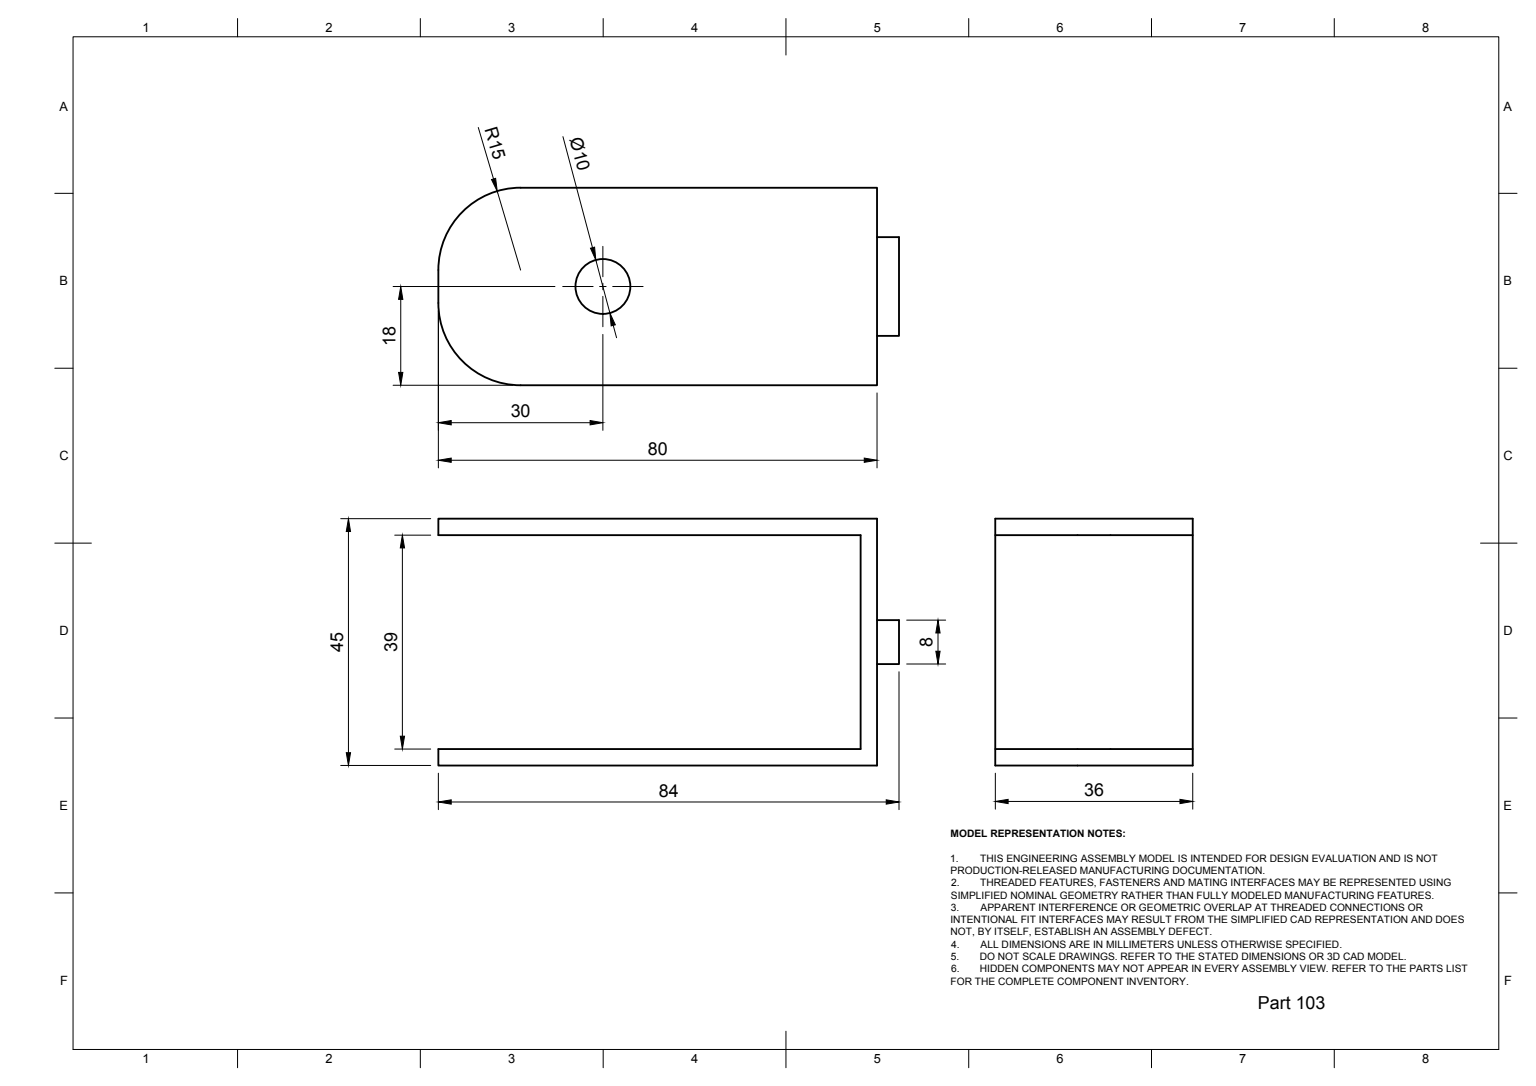
ISO-10303-21;
HEADER;
/* Generated by software containing ST-Developer
 * from STEP Tools, Inc. (www.steptools.com) 
 */

FILE_DESCRIPTION(
/* description */ (''),
/* implementation_level */ '2;1');

FILE_NAME(
/* name */ 'Part 103.step',
/* time_stamp */ '2026-10-07T11:02:43-07:00',
/* author */ (''),
/* organization */ (''),
/* preprocessor_version */ 'ST-DEVELOPER v20.2',
/* originating_system */ 'Autodesk Translation Framework v15.15.0.0',
/* authorisation */ '');

FILE_SCHEMA (('AUTOMOTIVE_DESIGN { 1 0 10303 214 3 1 1 }'));
ENDSEC;

DATA;
#10=MECHANICAL_DESIGN_GEOMETRIC_PRESENTATION_REPRESENTATION('',(#72),#5505);
#58=SHAPE_REPRESENTATION_RELATIONSHIP('SRR','None',#5543,#65);
#65=ADVANCED_BREP_SHAPE_REPRESENTATION('',(#79),#5504);
#72=STYLED_ITEM('',(#5587),#79);
#79=MANIFOLD_SOLID_BREP('Body1',#3299);
#108=FACE_BOUND('',#577,.T.);
#109=FACE_BOUND('',#579,.T.);
#110=FACE_BOUND('',#582,.T.);
#111=FACE_BOUND('',#584,.T.);
#112=FACE_BOUND('',#586,.T.);
#147=CYLINDRICAL_SURFACE('',#3629,15.);
#148=CYLINDRICAL_SURFACE('',#3630,15.);
#149=CYLINDRICAL_SURFACE('',#3631,15.);
#150=CYLINDRICAL_SURFACE('',#3632,15.);
#151=CYLINDRICAL_SURFACE('',#3633,5.);
#152=CYLINDRICAL_SURFACE('',#3634,5.);
#224=CIRCLE('',#3604,15.);
#225=CIRCLE('',#3605,15.);
#226=CIRCLE('',#3606,5.);
#227=CIRCLE('',#3608,15.);
#228=CIRCLE('',#3609,15.);
#229=CIRCLE('',#3610,5.);
#230=CIRCLE('',#3613,15.);
#231=CIRCLE('',#3614,15.);
#232=CIRCLE('',#3615,5.);
#233=CIRCLE('',#3617,15.);
#234=CIRCLE('',#3618,15.);
#235=CIRCLE('',#3619,5.);
#381=FACE_OUTER_BOUND('',#575,.T.);
#382=FACE_OUTER_BOUND('',#576,.T.);
#383=FACE_OUTER_BOUND('',#578,.T.);
#384=FACE_OUTER_BOUND('',#580,.T.);
#385=FACE_OUTER_BOUND('',#581,.T.);
#386=FACE_OUTER_BOUND('',#583,.T.);
#387=FACE_OUTER_BOUND('',#585,.T.);
#388=FACE_OUTER_BOUND('',#587,.T.);
#389=FACE_OUTER_BOUND('',#588,.T.);
#390=FACE_OUTER_BOUND('',#589,.T.);
#391=FACE_OUTER_BOUND('',#590,.T.);
#392=FACE_OUTER_BOUND('',#591,.T.);
#393=FACE_OUTER_BOUND('',#592,.T.);
#394=FACE_OUTER_BOUND('',#593,.T.);
#395=FACE_OUTER_BOUND('',#594,.T.);
#396=FACE_OUTER_BOUND('',#595,.T.);
#397=FACE_OUTER_BOUND('',#596,.T.);
#398=FACE_OUTER_BOUND('',#597,.T.);
#399=FACE_OUTER_BOUND('',#598,.T.);
#400=FACE_OUTER_BOUND('',#599,.T.);
#401=FACE_OUTER_BOUND('',#600,.T.);
#575=EDGE_LOOP('',(#2894,#2895,#2896,#2897));
#576=EDGE_LOOP('',(#2898,#2899,#2900,#2901,#2902,#2903));
#577=EDGE_LOOP('',(#2904));
#578=EDGE_LOOP('',(#2905,#2906,#2907,#2908,#2909,#2910));
#579=EDGE_LOOP('',(#2911));
#580=EDGE_LOOP('',(#2912,#2913,#2914,#2915));
#581=EDGE_LOOP('',(#2916,#2917,#2918,#2919,#2920,#2921));
#582=EDGE_LOOP('',(#2922));
#583=EDGE_LOOP('',(#2923,#2924,#2925,#2926,#2927,#2928));
#584=EDGE_LOOP('',(#2929));
#585=EDGE_LOOP('',(#2930,#2931,#2932,#2933));
#586=EDGE_LOOP('',(#2934,#2935,#2936,#2937));
#587=EDGE_LOOP('',(#2938,#2939,#2940,#2941,#2942,#2943,#2944,#2945));
#588=EDGE_LOOP('',(#2946,#2947,#2948,#2949,#2950,#2951,#2952,#2953));
#589=EDGE_LOOP('',(#2954,#2955,#2956,#2957));
#590=EDGE_LOOP('',(#2958,#2959,#2960,#2961));
#591=EDGE_LOOP('',(#2962,#2963,#2964,#2965));
#592=EDGE_LOOP('',(#2966,#2967,#2968,#2969));
#593=EDGE_LOOP('',(#2970,#2971,#2972,#2973));
#594=EDGE_LOOP('',(#2974,#2975,#2976,#2977));
#595=EDGE_LOOP('',(#2978,#2979,#2980,#2981));
#596=EDGE_LOOP('',(#2982,#2983,#2984,#2985));
#597=EDGE_LOOP('',(#2986,#2987,#2988,#2989));
#598=EDGE_LOOP('',(#2990,#2991,#2992,#2993));
#599=EDGE_LOOP('',(#2994,#2995,#2996,#2997));
#600=EDGE_LOOP('',(#2998,#2999,#3000,#3001));
#929=LINE('',#5370,#1299);
#930=LINE('',#5372,#1300);
#931=LINE('',#5374,#1301);
#932=LINE('',#5375,#1302);
#933=LINE('',#5379,#1303);
#934=LINE('',#5384,#1304);
#935=LINE('',#5385,#1305);
#936=LINE('',#5393,#1306);
#937=LINE('',#5395,#1307);
#938=LINE('',#5397,#1308);
#939=LINE('',#5400,#1309);
#940=LINE('',#5405,#1310);
#941=LINE('',#5407,#1311);
#942=LINE('',#5408,#1312);
#943=LINE('',#5413,#1313);
#944=LINE('',#5415,#1314);
#945=LINE('',#5417,#1315);
#946=LINE('',#5427,#1316);
#947=LINE('',#5429,#1317);
#948=LINE('',#5430,#1318);
#949=LINE('',#5434,#1319);
#950=LINE('',#5435,#1320);
#951=LINE('',#5438,#1321);
#952=LINE('',#5440,#1322);
#953=LINE('',#5442,#1323);
#954=LINE('',#5443,#1324);
#955=LINE('',#5445,#1325);
#956=LINE('',#5446,#1326);
#957=LINE('',#5447,#1327);
#958=LINE('',#5449,#1328);
#959=LINE('',#5450,#1329);
#960=LINE('',#5451,#1330);
#961=LINE('',#5455,#1331);
#962=LINE('',#5457,#1332);
#963=LINE('',#5458,#1333);
#964=LINE('',#5461,#1334);
#965=LINE('',#5462,#1335);
#966=LINE('',#5465,#1336);
#967=LINE('',#5466,#1337);
#968=LINE('',#5468,#1338);
#969=LINE('',#5475,#1339);
#970=LINE('',#5477,#1340);
#1299=VECTOR('',#4423,1000.);
#1300=VECTOR('',#4424,1000.);
#1301=VECTOR('',#4425,1000.);
#1302=VECTOR('',#4426,1000.);
#1303=VECTOR('',#4429,1000.);
#1304=VECTOR('',#4434,1000.);
#1305=VECTOR('',#4435,1000.);
#1306=VECTOR('',#4442,1000.);
#1307=VECTOR('',#4443,1000.);
#1308=VECTOR('',#4444,1000.);
#1309=VECTOR('',#4447,1000.);
#1310=VECTOR('',#4452,1000.);
#1311=VECTOR('',#4453,1000.);
#1312=VECTOR('',#4454,1000.);
#1313=VECTOR('',#4459,1000.);
#1314=VECTOR('',#4460,1000.);
#1315=VECTOR('',#4461,1000.);
#1316=VECTOR('',#4472,1000.);
#1317=VECTOR('',#4473,1000.);
#1318=VECTOR('',#4474,1000.);
#1319=VECTOR('',#4479,1000.);
#1320=VECTOR('',#4480,1000.);
#1321=VECTOR('',#4481,1000.);
#1322=VECTOR('',#4482,1000.);
#1323=VECTOR('',#4483,1000.);
#1324=VECTOR('',#4484,1000.);
#1325=VECTOR('',#4487,1000.);
#1326=VECTOR('',#4488,1000.);
#1327=VECTOR('',#4489,1000.);
#1328=VECTOR('',#4492,1000.);
#1329=VECTOR('',#4493,1000.);
#1330=VECTOR('',#4494,1000.);
#1331=VECTOR('',#4499,1000.);
#1332=VECTOR('',#4500,1000.);
#1333=VECTOR('',#4501,1000.);
#1334=VECTOR('',#4504,1000.);
#1335=VECTOR('',#4505,1000.);
#1336=VECTOR('',#4508,1000.);
#1337=VECTOR('',#4509,1000.);
#1338=VECTOR('',#4512,1000.);
#1339=VECTOR('',#4525,5.);
#1340=VECTOR('',#4528,5.);
#1607=VERTEX_POINT('',#5368);
#1608=VERTEX_POINT('',#5369);
#1609=VERTEX_POINT('',#5371);
#1610=VERTEX_POINT('',#5373);
#1611=VERTEX_POINT('',#5377);
#1612=VERTEX_POINT('',#5378);
#1613=VERTEX_POINT('',#5381);
#1614=VERTEX_POINT('',#5383);
#1615=VERTEX_POINT('',#5386);
#1616=VERTEX_POINT('',#5389);
#1617=VERTEX_POINT('',#5390);
#1618=VERTEX_POINT('',#5392);
#1619=VERTEX_POINT('',#5394);
#1620=VERTEX_POINT('',#5396);
#1621=VERTEX_POINT('',#5398);
#1622=VERTEX_POINT('',#5401);
#1623=VERTEX_POINT('',#5404);
#1624=VERTEX_POINT('',#5406);
#1625=VERTEX_POINT('',#5410);
#1626=VERTEX_POINT('',#5412);
#1627=VERTEX_POINT('',#5414);
#1628=VERTEX_POINT('',#5416);
#1629=VERTEX_POINT('',#5419);
#1630=VERTEX_POINT('',#5422);
#1631=VERTEX_POINT('',#5424);
#1632=VERTEX_POINT('',#5426);
#1633=VERTEX_POINT('',#5428);
#1634=VERTEX_POINT('',#5431);
#1635=VERTEX_POINT('',#5436);
#1636=VERTEX_POINT('',#5437);
#1637=VERTEX_POINT('',#5439);
#1638=VERTEX_POINT('',#5441);
#1639=VERTEX_POINT('',#5454);
#1640=VERTEX_POINT('',#5456);
#1641=VERTEX_POINT('',#5460);
#1642=VERTEX_POINT('',#5464);
#2042=EDGE_CURVE('',#1607,#1608,#929,.T.);
#2043=EDGE_CURVE('',#1608,#1609,#930,.T.);
#2044=EDGE_CURVE('',#1610,#1609,#931,.T.);
#2045=EDGE_CURVE('',#1607,#1610,#932,.T.);
#2046=EDGE_CURVE('',#1611,#1612,#933,.T.);
#2047=EDGE_CURVE('',#1611,#1610,#224,.T.);
#2048=EDGE_CURVE('',#1609,#1613,#225,.T.);
#2049=EDGE_CURVE('',#1613,#1614,#934,.T.);
#2050=EDGE_CURVE('',#1612,#1614,#935,.T.);
#2051=EDGE_CURVE('',#1615,#1615,#226,.T.);
#2052=EDGE_CURVE('',#1616,#1617,#227,.T.);
#2053=EDGE_CURVE('',#1616,#1618,#936,.T.);
#2054=EDGE_CURVE('',#1618,#1619,#937,.T.);
#2055=EDGE_CURVE('',#1620,#1619,#938,.T.);
#2056=EDGE_CURVE('',#1621,#1620,#228,.T.);
#2057=EDGE_CURVE('',#1617,#1621,#939,.T.);
#2058=EDGE_CURVE('',#1622,#1622,#229,.T.);
#2059=EDGE_CURVE('',#1621,#1623,#940,.T.);
#2060=EDGE_CURVE('',#1624,#1623,#941,.T.);
#2061=EDGE_CURVE('',#1617,#1624,#942,.T.);
#2062=EDGE_CURVE('',#1607,#1625,#230,.T.);
#2063=EDGE_CURVE('',#1626,#1625,#943,.T.);
#2064=EDGE_CURVE('',#1627,#1626,#944,.T.);
#2065=EDGE_CURVE('',#1628,#1627,#945,.T.);
#2066=EDGE_CURVE('',#1628,#1608,#231,.T.);
#2067=EDGE_CURVE('',#1629,#1629,#232,.T.);
#2068=EDGE_CURVE('',#1624,#1630,#233,.T.);
#2069=EDGE_CURVE('',#1631,#1623,#234,.T.);
#2070=EDGE_CURVE('',#1631,#1632,#946,.T.);
#2071=EDGE_CURVE('',#1632,#1633,#947,.T.);
#2072=EDGE_CURVE('',#1633,#1630,#948,.T.);
#2073=EDGE_CURVE('',#1634,#1634,#235,.T.);
#2074=EDGE_CURVE('',#1614,#1619,#949,.T.);
#2075=EDGE_CURVE('',#1612,#1618,#950,.T.);
#2076=EDGE_CURVE('',#1635,#1636,#951,.T.);
#2077=EDGE_CURVE('',#1635,#1637,#952,.T.);
#2078=EDGE_CURVE('',#1637,#1638,#953,.T.);
#2079=EDGE_CURVE('',#1636,#1638,#954,.T.);
#2080=EDGE_CURVE('',#1620,#1631,#955,.T.);
#2081=EDGE_CURVE('',#1628,#1613,#956,.T.);
#2082=EDGE_CURVE('',#1632,#1627,#957,.T.);
#2083=EDGE_CURVE('',#1616,#1630,#958,.T.);
#2084=EDGE_CURVE('',#1626,#1633,#959,.T.);
#2085=EDGE_CURVE('',#1625,#1611,#960,.T.);
#2086=EDGE_CURVE('',#1639,#1636,#961,.T.);
#2087=EDGE_CURVE('',#1640,#1639,#962,.T.);
#2088=EDGE_CURVE('',#1640,#1635,#963,.T.);
#2089=EDGE_CURVE('',#1641,#1638,#964,.T.);
#2090=EDGE_CURVE('',#1639,#1641,#965,.T.);
#2091=EDGE_CURVE('',#1642,#1637,#966,.T.);
#2092=EDGE_CURVE('',#1642,#1641,#967,.T.);
#2093=EDGE_CURVE('',#1640,#1642,#968,.T.);
#2094=EDGE_CURVE('',#1622,#1634,#969,.T.);
#2095=EDGE_CURVE('',#1629,#1615,#970,.T.);
#2894=ORIENTED_EDGE('',*,*,#2042,.T.);
#2895=ORIENTED_EDGE('',*,*,#2043,.T.);
#2896=ORIENTED_EDGE('',*,*,#2044,.F.);
#2897=ORIENTED_EDGE('',*,*,#2045,.F.);
#2898=ORIENTED_EDGE('',*,*,#2046,.F.);
#2899=ORIENTED_EDGE('',*,*,#2047,.T.);
#2900=ORIENTED_EDGE('',*,*,#2044,.T.);
#2901=ORIENTED_EDGE('',*,*,#2048,.T.);
#2902=ORIENTED_EDGE('',*,*,#2049,.T.);
#2903=ORIENTED_EDGE('',*,*,#2050,.F.);
#2904=ORIENTED_EDGE('',*,*,#2051,.F.);
#2905=ORIENTED_EDGE('',*,*,#2052,.F.);
#2906=ORIENTED_EDGE('',*,*,#2053,.T.);
#2907=ORIENTED_EDGE('',*,*,#2054,.T.);
#2908=ORIENTED_EDGE('',*,*,#2055,.F.);
#2909=ORIENTED_EDGE('',*,*,#2056,.F.);
#2910=ORIENTED_EDGE('',*,*,#2057,.F.);
#2911=ORIENTED_EDGE('',*,*,#2058,.T.);
#2912=ORIENTED_EDGE('',*,*,#2057,.T.);
#2913=ORIENTED_EDGE('',*,*,#2059,.T.);
#2914=ORIENTED_EDGE('',*,*,#2060,.F.);
#2915=ORIENTED_EDGE('',*,*,#2061,.F.);
#2916=ORIENTED_EDGE('',*,*,#2042,.F.);
#2917=ORIENTED_EDGE('',*,*,#2062,.T.);
#2918=ORIENTED_EDGE('',*,*,#2063,.F.);
#2919=ORIENTED_EDGE('',*,*,#2064,.F.);
#2920=ORIENTED_EDGE('',*,*,#2065,.F.);
#2921=ORIENTED_EDGE('',*,*,#2066,.T.);
#2922=ORIENTED_EDGE('',*,*,#2067,.F.);
#2923=ORIENTED_EDGE('',*,*,#2068,.F.);
#2924=ORIENTED_EDGE('',*,*,#2060,.T.);
#2925=ORIENTED_EDGE('',*,*,#2069,.F.);
#2926=ORIENTED_EDGE('',*,*,#2070,.T.);
#2927=ORIENTED_EDGE('',*,*,#2071,.T.);
#2928=ORIENTED_EDGE('',*,*,#2072,.T.);
#2929=ORIENTED_EDGE('',*,*,#2073,.T.);
#2930=ORIENTED_EDGE('',*,*,#2050,.T.);
#2931=ORIENTED_EDGE('',*,*,#2074,.T.);
#2932=ORIENTED_EDGE('',*,*,#2054,.F.);
#2933=ORIENTED_EDGE('',*,*,#2075,.F.);
#2934=ORIENTED_EDGE('',*,*,#2076,.F.);
#2935=ORIENTED_EDGE('',*,*,#2077,.T.);
#2936=ORIENTED_EDGE('',*,*,#2078,.T.);
#2937=ORIENTED_EDGE('',*,*,#2079,.F.);
#2938=ORIENTED_EDGE('',*,*,#2080,.F.);
#2939=ORIENTED_EDGE('',*,*,#2055,.T.);
#2940=ORIENTED_EDGE('',*,*,#2074,.F.);
#2941=ORIENTED_EDGE('',*,*,#2049,.F.);
#2942=ORIENTED_EDGE('',*,*,#2081,.F.);
#2943=ORIENTED_EDGE('',*,*,#2065,.T.);
#2944=ORIENTED_EDGE('',*,*,#2082,.F.);
#2945=ORIENTED_EDGE('',*,*,#2070,.F.);
#2946=ORIENTED_EDGE('',*,*,#2053,.F.);
#2947=ORIENTED_EDGE('',*,*,#2083,.T.);
#2948=ORIENTED_EDGE('',*,*,#2072,.F.);
#2949=ORIENTED_EDGE('',*,*,#2084,.F.);
#2950=ORIENTED_EDGE('',*,*,#2063,.T.);
#2951=ORIENTED_EDGE('',*,*,#2085,.T.);
#2952=ORIENTED_EDGE('',*,*,#2046,.T.);
#2953=ORIENTED_EDGE('',*,*,#2075,.T.);
#2954=ORIENTED_EDGE('',*,*,#2082,.T.);
#2955=ORIENTED_EDGE('',*,*,#2064,.T.);
#2956=ORIENTED_EDGE('',*,*,#2084,.T.);
#2957=ORIENTED_EDGE('',*,*,#2071,.F.);
#2958=ORIENTED_EDGE('',*,*,#2076,.T.);
#2959=ORIENTED_EDGE('',*,*,#2086,.F.);
#2960=ORIENTED_EDGE('',*,*,#2087,.F.);
#2961=ORIENTED_EDGE('',*,*,#2088,.T.);
#2962=ORIENTED_EDGE('',*,*,#2079,.T.);
#2963=ORIENTED_EDGE('',*,*,#2089,.F.);
#2964=ORIENTED_EDGE('',*,*,#2090,.F.);
#2965=ORIENTED_EDGE('',*,*,#2086,.T.);
#2966=ORIENTED_EDGE('',*,*,#2078,.F.);
#2967=ORIENTED_EDGE('',*,*,#2091,.F.);
#2968=ORIENTED_EDGE('',*,*,#2092,.T.);
#2969=ORIENTED_EDGE('',*,*,#2089,.T.);
#2970=ORIENTED_EDGE('',*,*,#2077,.F.);
#2971=ORIENTED_EDGE('',*,*,#2088,.F.);
#2972=ORIENTED_EDGE('',*,*,#2093,.T.);
#2973=ORIENTED_EDGE('',*,*,#2091,.T.);
#2974=ORIENTED_EDGE('',*,*,#2087,.T.);
#2975=ORIENTED_EDGE('',*,*,#2090,.T.);
#2976=ORIENTED_EDGE('',*,*,#2092,.F.);
#2977=ORIENTED_EDGE('',*,*,#2093,.F.);
#2978=ORIENTED_EDGE('',*,*,#2056,.T.);
#2979=ORIENTED_EDGE('',*,*,#2080,.T.);
#2980=ORIENTED_EDGE('',*,*,#2069,.T.);
#2981=ORIENTED_EDGE('',*,*,#2059,.F.);
#2982=ORIENTED_EDGE('',*,*,#2052,.T.);
#2983=ORIENTED_EDGE('',*,*,#2061,.T.);
#2984=ORIENTED_EDGE('',*,*,#2068,.T.);
#2985=ORIENTED_EDGE('',*,*,#2083,.F.);
#2986=ORIENTED_EDGE('',*,*,#2081,.T.);
#2987=ORIENTED_EDGE('',*,*,#2048,.F.);
#2988=ORIENTED_EDGE('',*,*,#2043,.F.);
#2989=ORIENTED_EDGE('',*,*,#2066,.F.);
#2990=ORIENTED_EDGE('',*,*,#2045,.T.);
#2991=ORIENTED_EDGE('',*,*,#2047,.F.);
#2992=ORIENTED_EDGE('',*,*,#2085,.F.);
#2993=ORIENTED_EDGE('',*,*,#2062,.F.);
#2994=ORIENTED_EDGE('',*,*,#2058,.F.);
#2995=ORIENTED_EDGE('',*,*,#2094,.T.);
#2996=ORIENTED_EDGE('',*,*,#2073,.F.);
#2997=ORIENTED_EDGE('',*,*,#2094,.F.);
#2998=ORIENTED_EDGE('',*,*,#2067,.T.);
#2999=ORIENTED_EDGE('',*,*,#2095,.T.);
#3000=ORIENTED_EDGE('',*,*,#2051,.T.);
#3001=ORIENTED_EDGE('',*,*,#2095,.F.);
#3112=PLANE('',#3602);
#3113=PLANE('',#3603);
#3114=PLANE('',#3607);
#3115=PLANE('',#3611);
#3116=PLANE('',#3612);
#3117=PLANE('',#3616);
#3118=PLANE('',#3620);
#3119=PLANE('',#3621);
#3120=PLANE('',#3622);
#3121=PLANE('',#3623);
#3122=PLANE('',#3624);
#3123=PLANE('',#3625);
#3124=PLANE('',#3626);
#3125=PLANE('',#3627);
#3126=PLANE('',#3628);
#3272=ADVANCED_FACE('',(#381),#3112,.T.);
#3273=ADVANCED_FACE('',(#382,#108),#3113,.T.);
#3274=ADVANCED_FACE('',(#383,#109),#3114,.F.);
#3275=ADVANCED_FACE('',(#384),#3115,.T.);
#3276=ADVANCED_FACE('',(#385,#110),#3116,.T.);
#3277=ADVANCED_FACE('',(#386,#111),#3117,.F.);
#3278=ADVANCED_FACE('',(#387,#112),#3118,.F.);
#3279=ADVANCED_FACE('',(#388),#3119,.T.);
#3280=ADVANCED_FACE('',(#389),#3120,.F.);
#3281=ADVANCED_FACE('',(#390),#3121,.F.);
#3282=ADVANCED_FACE('',(#391),#3122,.F.);
#3283=ADVANCED_FACE('',(#392),#3123,.F.);
#3284=ADVANCED_FACE('',(#393),#3124,.T.);
#3285=ADVANCED_FACE('',(#394),#3125,.T.);
#3286=ADVANCED_FACE('',(#395),#3126,.T.);
#3287=ADVANCED_FACE('',(#396),#147,.T.);
#3288=ADVANCED_FACE('',(#397),#148,.T.);
#3289=ADVANCED_FACE('',(#398),#149,.T.);
#3290=ADVANCED_FACE('',(#399),#150,.T.);
#3291=ADVANCED_FACE('',(#400),#151,.F.);
#3292=ADVANCED_FACE('',(#401),#152,.F.);
#3299=CLOSED_SHELL('',(#3272,#3273,#3274,#3275,#3276,#3277,#3278,#3279,
#3280,#3281,#3282,#3283,#3284,#3285,#3286,#3287,#3288,#3289,#3290,#3291,
#3292));
#3601=AXIS2_PLACEMENT_3D('',#5366,#4419,#4420);
#3602=AXIS2_PLACEMENT_3D('',#5367,#4421,#4422);
#3603=AXIS2_PLACEMENT_3D('',#5376,#4427,#4428);
#3604=AXIS2_PLACEMENT_3D('',#5380,#4430,#4431);
#3605=AXIS2_PLACEMENT_3D('',#5382,#4432,#4433);
#3606=AXIS2_PLACEMENT_3D('',#5387,#4436,#4437);
#3607=AXIS2_PLACEMENT_3D('',#5388,#4438,#4439);
#3608=AXIS2_PLACEMENT_3D('',#5391,#4440,#4441);
#3609=AXIS2_PLACEMENT_3D('',#5399,#4445,#4446);
#3610=AXIS2_PLACEMENT_3D('',#5402,#4448,#4449);
#3611=AXIS2_PLACEMENT_3D('',#5403,#4450,#4451);
#3612=AXIS2_PLACEMENT_3D('',#5409,#4455,#4456);
#3613=AXIS2_PLACEMENT_3D('',#5411,#4457,#4458);
#3614=AXIS2_PLACEMENT_3D('',#5418,#4462,#4463);
#3615=AXIS2_PLACEMENT_3D('',#5420,#4464,#4465);
#3616=AXIS2_PLACEMENT_3D('',#5421,#4466,#4467);
#3617=AXIS2_PLACEMENT_3D('',#5423,#4468,#4469);
#3618=AXIS2_PLACEMENT_3D('',#5425,#4470,#4471);
#3619=AXIS2_PLACEMENT_3D('',#5432,#4475,#4476);
#3620=AXIS2_PLACEMENT_3D('',#5433,#4477,#4478);
#3621=AXIS2_PLACEMENT_3D('',#5444,#4485,#4486);
#3622=AXIS2_PLACEMENT_3D('',#5448,#4490,#4491);
#3623=AXIS2_PLACEMENT_3D('',#5452,#4495,#4496);
#3624=AXIS2_PLACEMENT_3D('',#5453,#4497,#4498);
#3625=AXIS2_PLACEMENT_3D('',#5459,#4502,#4503);
#3626=AXIS2_PLACEMENT_3D('',#5463,#4506,#4507);
#3627=AXIS2_PLACEMENT_3D('',#5467,#4510,#4511);
#3628=AXIS2_PLACEMENT_3D('',#5469,#4513,#4514);
#3629=AXIS2_PLACEMENT_3D('',#5470,#4515,#4516);
#3630=AXIS2_PLACEMENT_3D('',#5471,#4517,#4518);
#3631=AXIS2_PLACEMENT_3D('',#5472,#4519,#4520);
#3632=AXIS2_PLACEMENT_3D('',#5473,#4521,#4522);
#3633=AXIS2_PLACEMENT_3D('',#5474,#4523,#4524);
#3634=AXIS2_PLACEMENT_3D('',#5476,#4526,#4527);
#4419=DIRECTION('axis',(0.,0.,1.));
#4420=DIRECTION('refdir',(1.,0.,0.));
#4421=DIRECTION('center_axis',(1.77035296021731E-31,1.,5.78241158658936E-16));
#4422=DIRECTION('ref_axis',(-1.,1.77035296021731E-31,1.02369094695133E-46));
#4423=DIRECTION('',(-1.09476442525376E-47,5.78241158658936E-16,-1.));
#4424=DIRECTION('',(-1.,1.77035296021731E-31,0.));
#4425=DIRECTION('',(1.02369094695133E-46,5.78241158658936E-16,-1.));
#4426=DIRECTION('',(-1.,1.77035296021731E-31,0.));
#4427=DIRECTION('center_axis',(-1.,1.77035296021731E-31,0.));
#4428=DIRECTION('ref_axis',(-1.77035296021731E-31,-1.,0.));
#4429=DIRECTION('',(-1.77035296021731E-31,-1.,-5.78241158658936E-16));
#4430=DIRECTION('center_axis',(-1.,1.77035296021731E-31,0.));
#4431=DIRECTION('ref_axis',(-1.77035296021731E-31,-1.,0.));
#4432=DIRECTION('center_axis',(-1.,1.77035296021731E-31,0.));
#4433=DIRECTION('ref_axis',(-1.77035296021731E-31,-1.,0.));
#4434=DIRECTION('',(-1.77035296021731E-31,-1.,-5.78241158658936E-16));
#4435=DIRECTION('',(1.02369094695133E-46,5.78241158658936E-16,-1.));
#4436=DIRECTION('center_axis',(-1.,1.77035296021731E-31,0.));
#4437=DIRECTION('ref_axis',(-1.77035296021731E-31,-1.,0.));
#4438=DIRECTION('center_axis',(-1.,1.77035296021731E-31,0.));
#4439=DIRECTION('ref_axis',(-1.77035296021731E-31,-1.,0.));
#4440=DIRECTION('center_axis',(-1.,1.77035296021731E-31,0.));
#4441=DIRECTION('ref_axis',(-1.77035296021731E-31,-1.,0.));
#4442=DIRECTION('',(-1.77035296021731E-31,-1.,-5.78241158658936E-16));
#4443=DIRECTION('',(1.02369094695133E-46,5.78241158658936E-16,-1.));
#4444=DIRECTION('',(-1.77035296021731E-31,-1.,-5.78241158658936E-16));
#4445=DIRECTION('center_axis',(-1.,1.77035296021731E-31,0.));
#4446=DIRECTION('ref_axis',(-1.77035296021731E-31,-1.,0.));
#4447=DIRECTION('',(1.02369094695133E-46,5.78241158658936E-16,-1.));
#4448=DIRECTION('center_axis',(-1.,1.77035296021731E-31,0.));
#4449=DIRECTION('ref_axis',(-1.77035296021731E-31,-1.,0.));
#4450=DIRECTION('center_axis',(1.77035296021731E-31,1.,5.78241158658936E-16));
#4451=DIRECTION('ref_axis',(-1.,1.77035296021731E-31,1.02369094695133E-46));
#4452=DIRECTION('',(-1.,1.77035296021731E-31,0.));
#4453=DIRECTION('',(2.18952885050752E-47,5.78241158658936E-16,-1.));
#4454=DIRECTION('',(-1.,1.77035296021731E-31,0.));
#4455=DIRECTION('center_axis',(1.,1.34933644236765E-16,7.80241867855395E-32));
#4456=DIRECTION('ref_axis',(-1.34933644236765E-16,1.,3.27983892575899E-64));
#4457=DIRECTION('center_axis',(1.,1.34933644236765E-16,7.80241867855395E-32));
#4458=DIRECTION('ref_axis',(-1.34933644236765E-16,1.,3.27983892575899E-64));
#4459=DIRECTION('',(-1.34933644236765E-16,1.,5.78241158658936E-16));
#4460=DIRECTION('',(1.51929083932157E-62,-5.78241158658936E-16,1.));
#4461=DIRECTION('',(1.34933644236765E-16,-1.,-5.78241158658936E-16));
#4462=DIRECTION('center_axis',(1.,1.34933644236765E-16,7.80241867855395E-32));
#4463=DIRECTION('ref_axis',(-1.34933644236765E-16,1.,3.27983892575899E-64));
#4464=DIRECTION('center_axis',(1.,1.34933644236765E-16,7.80241867855395E-32));
#4465=DIRECTION('ref_axis',(-1.34933644236765E-16,1.,3.27983892575899E-64));
#4466=DIRECTION('center_axis',(1.,3.20467405062316E-16,1.85307443615657E-31));
#4467=DIRECTION('ref_axis',(-3.20467405062316E-16,1.,4.27650648726681E-63));
#4468=DIRECTION('center_axis',(1.,3.20467405062316E-16,1.85307443615657E-31));
#4469=DIRECTION('ref_axis',(-3.20467405062316E-16,1.,4.27650648726681E-63));
#4470=DIRECTION('center_axis',(1.,3.20467405062316E-16,1.85307443615657E-31));
#4471=DIRECTION('ref_axis',(-3.20467405062316E-16,1.,4.27650648726681E-63));
#4472=DIRECTION('',(3.20467405062316E-16,-1.,-5.78241158658936E-16));
#4473=DIRECTION('',(1.51929083932157E-62,-5.78241158658936E-16,1.));
#4474=DIRECTION('',(-3.20467405062316E-16,1.,5.78241158658936E-16));
#4475=DIRECTION('center_axis',(1.,3.20467405062316E-16,1.85307443615657E-31));
#4476=DIRECTION('ref_axis',(-3.20467405062316E-16,1.,4.27650648726681E-63));
#4477=DIRECTION('center_axis',(1.77035296021731E-31,1.,5.78241158658936E-16));
#4478=DIRECTION('ref_axis',(-1.,1.77035296021731E-31,1.02369094695133E-46));
#4479=DIRECTION('',(1.,-1.77035296021731E-31,-1.02369094695133E-46));
#4480=DIRECTION('',(1.,-1.77035296021731E-31,-1.02369094695133E-46));
#4481=DIRECTION('',(1.02369094695133E-46,5.78241158658936E-16,-1.));
#4482=DIRECTION('',(1.,-1.77035296021731E-31,-1.02369094695133E-46));
#4483=DIRECTION('',(1.02369094695133E-46,5.78241158658936E-16,-1.));
#4484=DIRECTION('',(1.,-1.77035296021731E-31,-1.02369094695133E-46));
#4485=DIRECTION('center_axis',(-1.51929083932157E-62,5.78241158658936E-16,
-1.));
#4486=DIRECTION('ref_axis',(0.,1.,5.78241158658936E-16));
#4487=DIRECTION('',(-1.,1.77035296021731E-31,0.));
#4488=DIRECTION('',(-1.,1.77035296021731E-31,0.));
#4489=DIRECTION('',(-1.,-8.7851649526921E-78,1.51929083932157E-62));
#4490=DIRECTION('center_axis',(-1.51929083932157E-62,5.78241158658936E-16,
-1.));
#4491=DIRECTION('ref_axis',(0.,1.,5.78241158658936E-16));
#4492=DIRECTION('',(-1.,1.77035296021731E-31,0.));
#4493=DIRECTION('',(1.,8.7851649526921E-78,-1.51929083932157E-62));
#4494=DIRECTION('',(-1.,1.77035296021731E-31,0.));
#4495=DIRECTION('center_axis',(-1.53655018820667E-93,-1.,-5.78241158658936E-16));
#4496=DIRECTION('ref_axis',(-4.01263672442025E-125,5.78241158658936E-16,
-1.));
#4497=DIRECTION('center_axis',(1.,-1.77035296021731E-31,0.));
#4498=DIRECTION('ref_axis',(1.77035296021731E-31,1.,0.));
#4499=DIRECTION('',(1.77035296021731E-31,1.,5.78241158658936E-16));
#4500=DIRECTION('',(1.02369094695133E-46,5.78241158658936E-16,-1.));
#4501=DIRECTION('',(1.77035296021731E-31,1.,5.78241158658936E-16));
#4502=DIRECTION('center_axis',(0.,-5.78241158658936E-16,1.));
#4503=DIRECTION('ref_axis',(0.,-1.,-5.78241158658936E-16));
#4504=DIRECTION('',(1.77035296021731E-31,1.,5.78241158658936E-16));
#4505=DIRECTION('',(1.,-1.77035296021731E-31,-1.02369094695133E-46));
#4506=DIRECTION('center_axis',(1.,-1.77035296021731E-31,0.));
#4507=DIRECTION('ref_axis',(1.77035296021731E-31,1.,0.));
#4508=DIRECTION('',(1.77035296021731E-31,1.,5.78241158658936E-16));
#4509=DIRECTION('',(1.02369094695133E-46,5.78241158658936E-16,-1.));
#4510=DIRECTION('center_axis',(0.,-5.78241158658936E-16,1.));
#4511=DIRECTION('ref_axis',(0.,-1.,-5.78241158658936E-16));
#4512=DIRECTION('',(1.,-1.77035296021731E-31,-1.02369094695133E-46));
#4513=DIRECTION('center_axis',(-1.77035296021731E-31,-1.,-5.78241158658936E-16));
#4514=DIRECTION('ref_axis',(1.,-1.77035296021731E-31,-1.02369094695133E-46));
#4515=DIRECTION('center_axis',(-1.,1.77035296021731E-31,0.));
#4516=DIRECTION('ref_axis',(-1.77035296021731E-31,-1.,0.));
#4517=DIRECTION('center_axis',(-1.,1.77035296021731E-31,0.));
#4518=DIRECTION('ref_axis',(-1.77035296021731E-31,-1.,0.));
#4519=DIRECTION('center_axis',(-1.,1.77035296021731E-31,0.));
#4520=DIRECTION('ref_axis',(-1.77035296021731E-31,-1.,0.));
#4521=DIRECTION('center_axis',(-1.,1.77035296021731E-31,0.));
#4522=DIRECTION('ref_axis',(-1.77035296021731E-31,-1.,0.));
#4523=DIRECTION('center_axis',(-1.,1.77035296021731E-31,0.));
#4524=DIRECTION('ref_axis',(-1.77035296021731E-31,-1.,0.));
#4525=DIRECTION('',(-1.,1.77035296021731E-31,0.));
#4526=DIRECTION('center_axis',(-1.,1.77035296021731E-31,0.));
#4527=DIRECTION('ref_axis',(-1.77035296021731E-31,-1.,0.));
#4528=DIRECTION('',(-1.,1.77035296021731E-31,0.));
#5366=CARTESIAN_POINT('',(0.,0.,0.));
#5367=CARTESIAN_POINT('Origin',(-32.,950.,107.));
#5368=CARTESIAN_POINT('',(-51.499999999999,950.,110.));
#5369=CARTESIAN_POINT('',(-51.5,950.,104.));
#5370=CARTESIAN_POINT('',(-51.5,950.,107.));
#5371=CARTESIAN_POINT('',(-54.5,950.,104.));
#5372=CARTESIAN_POINT('',(3079.10575317586,950.,104.));
#5373=CARTESIAN_POINT('',(-54.5,950.,110.));
#5374=CARTESIAN_POINT('',(-54.5,950.,107.));
#5375=CARTESIAN_POINT('',(3079.10575317586,950.,110.));
#5376=CARTESIAN_POINT('Origin',(-54.5,950.,107.));
#5377=CARTESIAN_POINT('',(-54.5,935.,125.));
#5378=CARTESIAN_POINT('',(-54.5,870.,125.));
#5379=CARTESIAN_POINT('',(-54.5,950.,125.));
#5380=CARTESIAN_POINT('Origin',(-54.5,935.,110.));
#5381=CARTESIAN_POINT('',(-54.5,935.,89.));
#5382=CARTESIAN_POINT('Origin',(-54.5,935.,104.));
#5383=CARTESIAN_POINT('',(-54.5,870.,89.));
#5384=CARTESIAN_POINT('',(-54.5,950.,89.));
#5385=CARTESIAN_POINT('',(-54.5,870.,107.));
#5386=CARTESIAN_POINT('',(-54.4999999999999,925.,107.));
#5387=CARTESIAN_POINT('Origin',(-54.5,920.,107.));
#5388=CARTESIAN_POINT('Origin',(-9.5,950.,107.));
#5389=CARTESIAN_POINT('',(-9.49999999999918,935.,125.));
#5390=CARTESIAN_POINT('',(-9.4999999999974,950.,110.));
#5391=CARTESIAN_POINT('Origin',(-9.5,935.,110.));
#5392=CARTESIAN_POINT('',(-9.5,870.,125.));
#5393=CARTESIAN_POINT('',(-9.5,950.,125.));
#5394=CARTESIAN_POINT('',(-9.5,870.,89.));
#5395=CARTESIAN_POINT('',(-9.5,870.,107.));
#5396=CARTESIAN_POINT('',(-9.49999999999918,935.,89.));
#5397=CARTESIAN_POINT('',(-9.5,950.,89.));
#5398=CARTESIAN_POINT('',(-9.4999999999974,950.,104.));
#5399=CARTESIAN_POINT('Origin',(-9.5,935.,104.));
#5400=CARTESIAN_POINT('',(-9.5,950.,107.));
#5401=CARTESIAN_POINT('',(-9.49999999999989,925.,107.));
#5402=CARTESIAN_POINT('Origin',(-9.5,920.,107.));
#5403=CARTESIAN_POINT('Origin',(-32.,950.,107.));
#5404=CARTESIAN_POINT('',(-12.4999999999993,950.,104.));
#5405=CARTESIAN_POINT('',(3079.10575317586,950.,104.));
#5406=CARTESIAN_POINT('',(-12.5000000000002,950.,110.));
#5407=CARTESIAN_POINT('',(-12.5,950.,107.));
#5408=CARTESIAN_POINT('',(3079.10575317586,950.,110.));
#5409=CARTESIAN_POINT('Origin',(-51.5,924.424490483128,86.));
#5410=CARTESIAN_POINT('',(-51.5,935.,125.));
#5411=CARTESIAN_POINT('Origin',(-51.5,935.,110.));
#5412=CARTESIAN_POINT('',(-51.5,873.,125.));
#5413=CARTESIAN_POINT('',(-51.5,924.424490483128,125.));
#5414=CARTESIAN_POINT('',(-51.5,873.,89.));
#5415=CARTESIAN_POINT('',(-51.5,873.,86.));
#5416=CARTESIAN_POINT('',(-51.499999999999,935.,89.));
#5417=CARTESIAN_POINT('',(-51.5,950.,89.));
#5418=CARTESIAN_POINT('Origin',(-51.5,935.,104.));
#5419=CARTESIAN_POINT('',(-51.5,925.,107.));
#5420=CARTESIAN_POINT('Origin',(-51.5,920.,107.));
#5421=CARTESIAN_POINT('Origin',(-12.5,924.424490483128,86.));
#5422=CARTESIAN_POINT('',(-12.4999999999993,935.,125.));
#5423=CARTESIAN_POINT('Origin',(-12.5000000000002,935.,110.));
#5424=CARTESIAN_POINT('',(-12.5000000000002,935.,89.));
#5425=CARTESIAN_POINT('Origin',(-12.5000000000002,935.,104.));
#5426=CARTESIAN_POINT('',(-12.5,873.,89.));
#5427=CARTESIAN_POINT('',(-12.5,950.,89.));
#5428=CARTESIAN_POINT('',(-12.5,873.,125.));
#5429=CARTESIAN_POINT('',(-12.5,873.,86.));
#5430=CARTESIAN_POINT('',(-12.5,924.424490483128,125.));
#5431=CARTESIAN_POINT('',(-12.5000000000002,925.,107.));
#5432=CARTESIAN_POINT('Origin',(-12.5000000000002,920.,107.));
#5433=CARTESIAN_POINT('Origin',(-32.,870.,107.));
#5434=CARTESIAN_POINT('',(-32.,870.,89.));
#5435=CARTESIAN_POINT('',(-32.,870.,125.));
#5436=CARTESIAN_POINT('',(-36.,870.,116.));
#5437=CARTESIAN_POINT('',(-36.,870.,98.));
#5438=CARTESIAN_POINT('',(-36.,870.,107.));
#5439=CARTESIAN_POINT('',(-28.,870.,116.));
#5440=CARTESIAN_POINT('',(-32.,870.,116.));
#5441=CARTESIAN_POINT('',(-28.,870.,98.));
#5442=CARTESIAN_POINT('',(-28.,870.,107.));
#5443=CARTESIAN_POINT('',(-32.,870.,98.));
#5444=CARTESIAN_POINT('Origin',(-32.,950.,89.));
#5445=CARTESIAN_POINT('',(3079.10575317586,935.,89.));
#5446=CARTESIAN_POINT('',(3079.10575317586,935.,89.));
#5447=CARTESIAN_POINT('',(-32.,873.,89.));
#5448=CARTESIAN_POINT('Origin',(-32.,950.,125.));
#5449=CARTESIAN_POINT('',(3079.10575317586,935.,125.));
#5450=CARTESIAN_POINT('',(-32.,873.,125.));
#5451=CARTESIAN_POINT('',(3079.10575317586,935.,125.));
#5452=CARTESIAN_POINT('Origin',(-32.,873.,86.));
#5453=CARTESIAN_POINT('Origin',(-36.,866.,107.));
#5454=CARTESIAN_POINT('',(-36.,866.,98.));
#5455=CARTESIAN_POINT('',(-36.,866.,98.));
#5456=CARTESIAN_POINT('',(-36.,866.,116.));
#5457=CARTESIAN_POINT('',(-36.,866.,107.));
#5458=CARTESIAN_POINT('',(-36.,866.,116.));
#5459=CARTESIAN_POINT('Origin',(-32.,866.,98.));
#5460=CARTESIAN_POINT('',(-28.,866.,98.));
#5461=CARTESIAN_POINT('',(-28.,866.,98.));
#5462=CARTESIAN_POINT('',(-32.,866.,98.));
#5463=CARTESIAN_POINT('Origin',(-28.,866.,107.));
#5464=CARTESIAN_POINT('',(-28.,866.,116.));
#5465=CARTESIAN_POINT('',(-28.,866.,116.));
#5466=CARTESIAN_POINT('',(-28.,866.,107.));
#5467=CARTESIAN_POINT('Origin',(-32.,866.,116.));
#5468=CARTESIAN_POINT('',(-32.,866.,116.));
#5469=CARTESIAN_POINT('Origin',(-32.,866.,107.));
#5470=CARTESIAN_POINT('Origin',(3079.10575317586,935.,104.));
#5471=CARTESIAN_POINT('Origin',(3079.10575317586,935.,110.));
#5472=CARTESIAN_POINT('Origin',(3079.10575317586,935.,104.));
#5473=CARTESIAN_POINT('Origin',(3079.10575317586,935.,110.));
#5474=CARTESIAN_POINT('Origin',(3065.02807175404,920.,107.));
#5475=CARTESIAN_POINT('',(3065.02807175404,925.,107.));
#5476=CARTESIAN_POINT('Origin',(3065.02807175404,920.,107.));
#5477=CARTESIAN_POINT('',(3065.02807175404,925.,107.));
#5495=UNCERTAINTY_MEASURE_WITH_UNIT(LENGTH_MEASURE(0.01),#5506,
'DISTANCE_ACCURACY_VALUE',
'Maximum model space distance between geometric entities at asserted c
onnectivities');
#5496=UNCERTAINTY_MEASURE_WITH_UNIT(LENGTH_MEASURE(0.01),#5506,
'DISTANCE_ACCURACY_VALUE',
'Maximum model space distance between geometric entities at asserted c
onnectivities');
#5504=(
GEOMETRIC_REPRESENTATION_CONTEXT(3)
GLOBAL_UNCERTAINTY_ASSIGNED_CONTEXT((#5495))
GLOBAL_UNIT_ASSIGNED_CONTEXT((#5506,#5508,#5509))
REPRESENTATION_CONTEXT('','3D')
);
#5505=(
GEOMETRIC_REPRESENTATION_CONTEXT(3)
GLOBAL_UNCERTAINTY_ASSIGNED_CONTEXT((#5496))
GLOBAL_UNIT_ASSIGNED_CONTEXT((#5506,#5508,#5509))
REPRESENTATION_CONTEXT('','3D')
);
#5506=(
LENGTH_UNIT()
NAMED_UNIT(*)
SI_UNIT(.MILLI.,.METRE.)
);
#5508=(
NAMED_UNIT(*)
PLANE_ANGLE_UNIT()
SI_UNIT($,.RADIAN.)
);
#5509=(
NAMED_UNIT(*)
SI_UNIT($,.STERADIAN.)
SOLID_ANGLE_UNIT()
);
#5517=SHAPE_DEFINITION_REPRESENTATION(#5525,#5543);
#5525=PRODUCT_DEFINITION_SHAPE('',$,#5552);
#5543=SHAPE_REPRESENTATION('',(#3601),#5504);
#5544=PRODUCT_DEFINITION_CONTEXT('part definition',#5570,'design');
#5552=PRODUCT_DEFINITION('2026-10-07-17-03-48-181','Part 103',#5560,#5544);
#5560=PRODUCT_DEFINITION_FORMATION('',$,#5579);
#5570=APPLICATION_CONTEXT(
'Core Data for Automotive Mechanical Design Process');
#5571=PRODUCT_CONTEXT('part definition',#5570,'mechanical');
#5579=PRODUCT('2026-10-07-17-03-48-181','Part 103','Part 103',(#5571));
#5587=PRESENTATION_STYLE_ASSIGNMENT((#5595));
#5595=SURFACE_STYLE_USAGE(.BOTH.,#5603);
#5603=SURFACE_SIDE_STYLE('',(#5611));
#5611=SURFACE_STYLE_FILL_AREA(#5619);
#5619=FILL_AREA_STYLE('Opaque(165,165,165)',(#5627));
#5627=FILL_AREA_STYLE_COLOUR('Opaque(165,165,165)',#5635);
#5635=COLOUR_RGB('Opaque(165,165,165)', 0.09019608, 0.27058824, 0.51372549);
ENDSEC;
END-ISO-10303-21;
